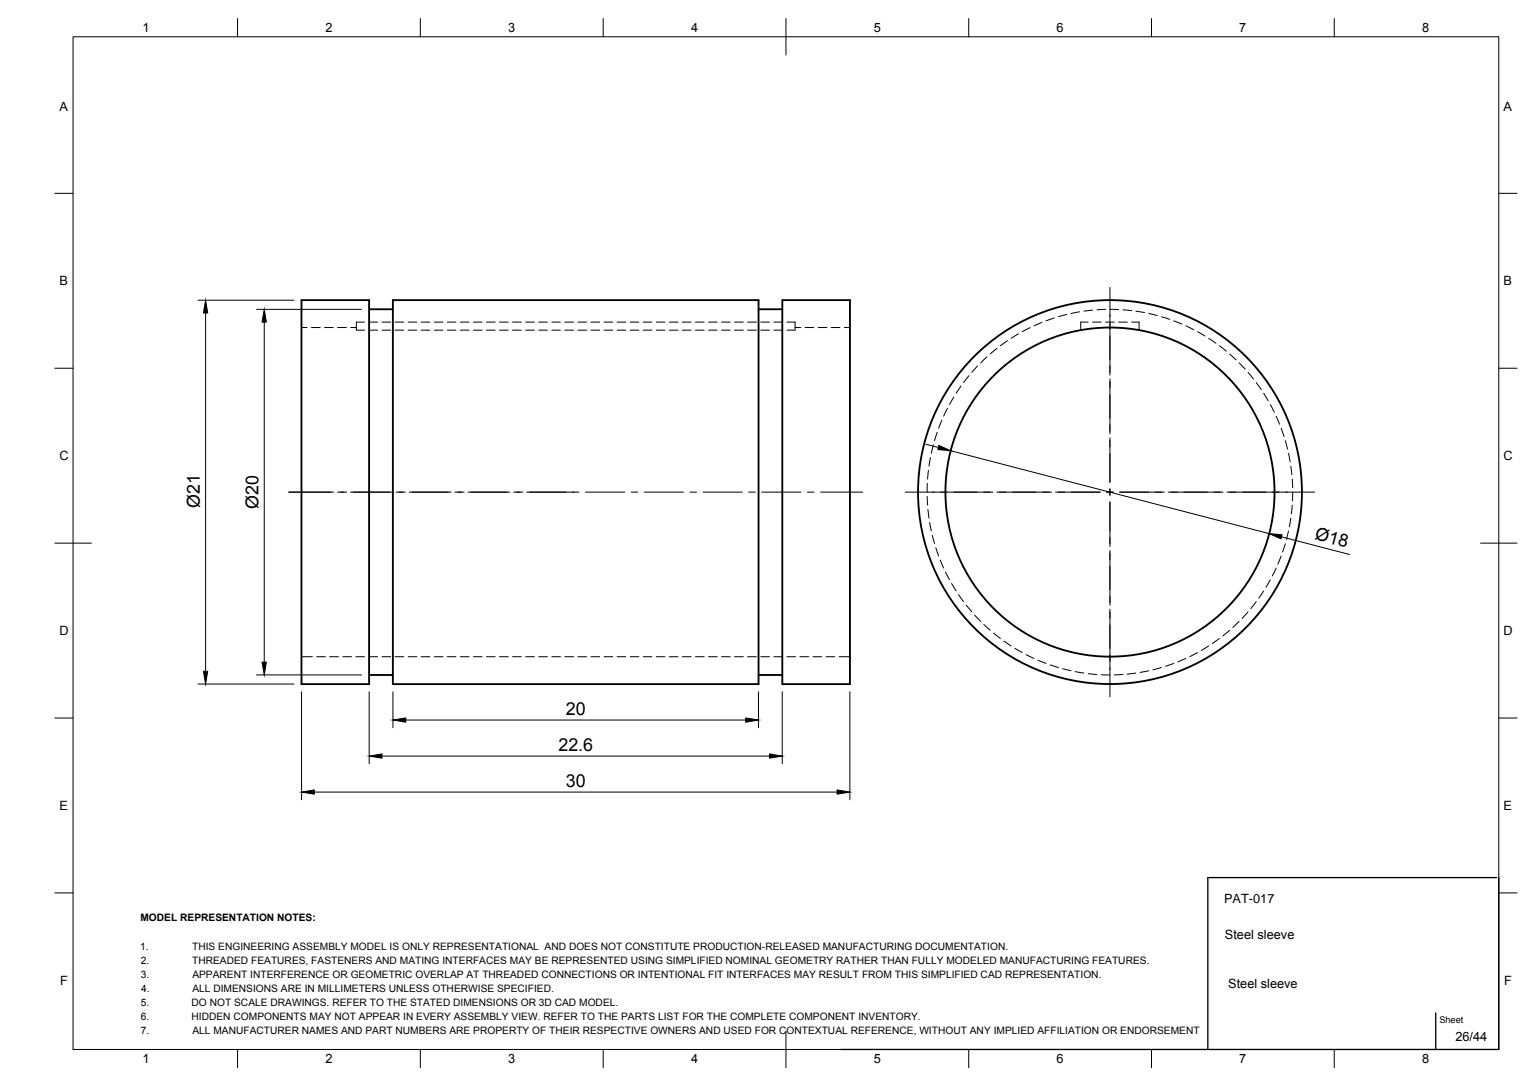
ISO-10303-21;
HEADER;
/* Generated by software containing ST-Developer
 * from STEP Tools, Inc. (www.steptools.com) 
 */

FILE_DESCRIPTION(
/* description */ ('Cam-and-follower valve demonstrator'),
/* implementation_level */ '2;1');

FILE_NAME(
/* name */ 'Steel sleeve.step',
/* time_stamp */ '2026-10-28T03:25:17-07:00',
/* author */ (''),
/* organization */ (''),
/* preprocessor_version */ 'ST-DEVELOPER v20.2',
/* originating_system */ 'Autodesk Translation Framework v15.17.0.0',
/* authorisation */ '');

FILE_SCHEMA (('AUTOMOTIVE_DESIGN { 1 0 10303 214 3 1 1 }'));
ENDSEC;

DATA;
#10=MECHANICAL_DESIGN_GEOMETRIC_PRESENTATION_REPRESENTATION('',(#437),#12896);
#358=SHAPE_REPRESENTATION_RELATIONSHIP('SRR','None',#13076,#394);
#394=ADVANCED_BREP_SHAPE_REPRESENTATION('',(#479),#12876);
#437=STYLED_ITEM('',(#13344),#479);
#479=MANIFOLD_SOLID_BREP('Body1',#6205);
#614=FACE_BOUND('',#1800,.T.);
#615=FACE_BOUND('',#1803,.T.);
#616=FACE_BOUND('',#1806,.T.);
#617=FACE_BOUND('',#1809,.T.);
#618=FACE_BOUND('',#1812,.T.);
#619=FACE_BOUND('',#1815,.T.);
#620=FACE_BOUND('',#1817,.T.);
#868=CIRCLE('',#7071,0.9);
#869=CIRCLE('',#7074,0.9);
#870=CIRCLE('',#7078,1.05);
#871=CIRCLE('',#7079,0.9);
#872=CIRCLE('',#7081,1.05);
#873=CIRCLE('',#7083,1.);
#874=CIRCLE('',#7085,1.);
#875=CIRCLE('',#7087,1.05);
#876=CIRCLE('',#7089,1.05);
#877=CIRCLE('',#7091,1.);
#878=CIRCLE('',#7093,1.);
#879=CIRCLE('',#7095,1.05);
#880=CIRCLE('',#7097,1.05);
#881=CIRCLE('',#7099,0.9);
#1052=CYLINDRICAL_SURFACE('',#7080,1.05);
#1053=CYLINDRICAL_SURFACE('',#7084,1.);
#1054=CYLINDRICAL_SURFACE('',#7088,1.05);
#1055=CYLINDRICAL_SURFACE('',#7092,1.);
#1056=CYLINDRICAL_SURFACE('',#7096,1.05);
#1057=CYLINDRICAL_SURFACE('',#7100,0.9);
#1307=FACE_OUTER_BOUND('',#1794,.T.);
#1308=FACE_OUTER_BOUND('',#1795,.T.);
#1309=FACE_OUTER_BOUND('',#1796,.T.);
#1310=FACE_OUTER_BOUND('',#1797,.T.);
#1311=FACE_OUTER_BOUND('',#1798,.T.);
#1312=FACE_OUTER_BOUND('',#1799,.T.);
#1313=FACE_OUTER_BOUND('',#1801,.T.);
#1314=FACE_OUTER_BOUND('',#1802,.T.);
#1315=FACE_OUTER_BOUND('',#1804,.T.);
#1316=FACE_OUTER_BOUND('',#1805,.T.);
#1317=FACE_OUTER_BOUND('',#1807,.T.);
#1318=FACE_OUTER_BOUND('',#1808,.T.);
#1319=FACE_OUTER_BOUND('',#1810,.T.);
#1320=FACE_OUTER_BOUND('',#1811,.T.);
#1321=FACE_OUTER_BOUND('',#1813,.T.);
#1322=FACE_OUTER_BOUND('',#1814,.T.);
#1323=FACE_OUTER_BOUND('',#1816,.T.);
#1794=EDGE_LOOP('',(#5017,#5018,#5019,#5020));
#1795=EDGE_LOOP('',(#5021,#5022,#5023,#5024));
#1796=EDGE_LOOP('',(#5025,#5026,#5027,#5028));
#1797=EDGE_LOOP('',(#5029,#5030,#5031,#5032));
#1798=EDGE_LOOP('',(#5033,#5034,#5035,#5036));
#1799=EDGE_LOOP('',(#5037));
#1800=EDGE_LOOP('',(#5038));
#1801=EDGE_LOOP('',(#5039,#5040,#5041,#5042));
#1802=EDGE_LOOP('',(#5043));
#1803=EDGE_LOOP('',(#5044));
#1804=EDGE_LOOP('',(#5045,#5046,#5047,#5048));
#1805=EDGE_LOOP('',(#5049));
#1806=EDGE_LOOP('',(#5050));
#1807=EDGE_LOOP('',(#5051,#5052,#5053,#5054));
#1808=EDGE_LOOP('',(#5055));
#1809=EDGE_LOOP('',(#5056));
#1810=EDGE_LOOP('',(#5057,#5058,#5059,#5060));
#1811=EDGE_LOOP('',(#5061));
#1812=EDGE_LOOP('',(#5062));
#1813=EDGE_LOOP('',(#5063,#5064,#5065,#5066));
#1814=EDGE_LOOP('',(#5067));
#1815=EDGE_LOOP('',(#5068));
#1816=EDGE_LOOP('',(#5069,#5070,#5071,#5072));
#1817=EDGE_LOOP('',(#5073,#5074,#5075,#5076));
#2232=LINE('',#12096,#2654);
#2233=LINE('',#12098,#2655);
#2234=LINE('',#12099,#2656);
#2235=LINE('',#12102,#2657);
#2236=LINE('',#12104,#2658);
#2237=LINE('',#12105,#2659);
#2238=LINE('',#12110,#2660);
#2239=LINE('',#12111,#2661);
#2240=LINE('',#12113,#2662);
#2241=LINE('',#12114,#2663);
#2242=LINE('',#12124,#2664);
#2243=LINE('',#12131,#2665);
#2244=LINE('',#12138,#2666);
#2245=LINE('',#12145,#2667);
#2246=LINE('',#12152,#2668);
#2247=LINE('',#12157,#2669);
#2654=VECTOR('',#8551,1.);
#2655=VECTOR('',#8552,1.);
#2656=VECTOR('',#8553,1.);
#2657=VECTOR('',#8556,1.);
#2658=VECTOR('',#8557,1.);
#2659=VECTOR('',#8558,1.);
#2660=VECTOR('',#8563,1.);
#2661=VECTOR('',#8564,1.);
#2662=VECTOR('',#8567,1.);
#2663=VECTOR('',#8568,1.);
#2664=VECTOR('',#8581,1.05);
#2665=VECTOR('',#8590,1.);
#2666=VECTOR('',#8599,1.05);
#2667=VECTOR('',#8608,1.);
#2668=VECTOR('',#8617,1.05);
#2669=VECTOR('',#8624,0.9);
#3153=VERTEX_POINT('',#12092);
#3154=VERTEX_POINT('',#12093);
#3155=VERTEX_POINT('',#12095);
#3156=VERTEX_POINT('',#12097);
#3157=VERTEX_POINT('',#12101);
#3158=VERTEX_POINT('',#12103);
#3159=VERTEX_POINT('',#12107);
#3160=VERTEX_POINT('',#12109);
#3161=VERTEX_POINT('',#12117);
#3162=VERTEX_POINT('',#12119);
#3163=VERTEX_POINT('',#12122);
#3164=VERTEX_POINT('',#12126);
#3165=VERTEX_POINT('',#12129);
#3166=VERTEX_POINT('',#12133);
#3167=VERTEX_POINT('',#12136);
#3168=VERTEX_POINT('',#12140);
#3169=VERTEX_POINT('',#12143);
#3170=VERTEX_POINT('',#12147);
#3171=VERTEX_POINT('',#12150);
#3172=VERTEX_POINT('',#12154);
#3805=EDGE_CURVE('',#3153,#3154,#868,.T.);
#3806=EDGE_CURVE('',#3155,#3153,#2232,.T.);
#3807=EDGE_CURVE('',#3156,#3155,#2233,.T.);
#3808=EDGE_CURVE('',#3154,#3156,#2234,.T.);
#3809=EDGE_CURVE('',#3154,#3157,#2235,.T.);
#3810=EDGE_CURVE('',#3158,#3156,#2236,.T.);
#3811=EDGE_CURVE('',#3158,#3157,#2237,.T.);
#3812=EDGE_CURVE('',#3157,#3159,#869,.T.);
#3813=EDGE_CURVE('',#3160,#3158,#2238,.T.);
#3814=EDGE_CURVE('',#3159,#3160,#2239,.T.);
#3815=EDGE_CURVE('',#3159,#3153,#2240,.T.);
#3816=EDGE_CURVE('',#3160,#3155,#2241,.T.);
#3817=EDGE_CURVE('',#3161,#3161,#870,.T.);
#3818=EDGE_CURVE('',#3162,#3162,#871,.T.);
#3819=EDGE_CURVE('',#3163,#3163,#872,.T.);
#3820=EDGE_CURVE('',#3163,#3161,#2242,.T.);
#3821=EDGE_CURVE('',#3164,#3164,#873,.T.);
#3822=EDGE_CURVE('',#3165,#3165,#874,.T.);
#3823=EDGE_CURVE('',#3165,#3164,#2243,.T.);
#3824=EDGE_CURVE('',#3166,#3166,#875,.T.);
#3825=EDGE_CURVE('',#3167,#3167,#876,.T.);
#3826=EDGE_CURVE('',#3167,#3166,#2244,.T.);
#3827=EDGE_CURVE('',#3168,#3168,#877,.T.);
#3828=EDGE_CURVE('',#3169,#3169,#878,.T.);
#3829=EDGE_CURVE('',#3169,#3168,#2245,.T.);
#3830=EDGE_CURVE('',#3170,#3170,#879,.T.);
#3831=EDGE_CURVE('',#3171,#3171,#880,.T.);
#3832=EDGE_CURVE('',#3171,#3170,#2246,.T.);
#3833=EDGE_CURVE('',#3172,#3172,#881,.T.);
#3834=EDGE_CURVE('',#3172,#3162,#2247,.T.);
#5017=ORIENTED_EDGE('',*,*,#3805,.F.);
#5018=ORIENTED_EDGE('',*,*,#3806,.F.);
#5019=ORIENTED_EDGE('',*,*,#3807,.F.);
#5020=ORIENTED_EDGE('',*,*,#3808,.F.);
#5021=ORIENTED_EDGE('',*,*,#3809,.F.);
#5022=ORIENTED_EDGE('',*,*,#3808,.T.);
#5023=ORIENTED_EDGE('',*,*,#3810,.F.);
#5024=ORIENTED_EDGE('',*,*,#3811,.T.);
#5025=ORIENTED_EDGE('',*,*,#3812,.F.);
#5026=ORIENTED_EDGE('',*,*,#3811,.F.);
#5027=ORIENTED_EDGE('',*,*,#3813,.F.);
#5028=ORIENTED_EDGE('',*,*,#3814,.F.);
#5029=ORIENTED_EDGE('',*,*,#3815,.F.);
#5030=ORIENTED_EDGE('',*,*,#3814,.T.);
#5031=ORIENTED_EDGE('',*,*,#3816,.T.);
#5032=ORIENTED_EDGE('',*,*,#3806,.T.);
#5033=ORIENTED_EDGE('',*,*,#3816,.F.);
#5034=ORIENTED_EDGE('',*,*,#3813,.T.);
#5035=ORIENTED_EDGE('',*,*,#3810,.T.);
#5036=ORIENTED_EDGE('',*,*,#3807,.T.);
#5037=ORIENTED_EDGE('',*,*,#3817,.F.);
#5038=ORIENTED_EDGE('',*,*,#3818,.T.);
#5039=ORIENTED_EDGE('',*,*,#3819,.F.);
#5040=ORIENTED_EDGE('',*,*,#3820,.T.);
#5041=ORIENTED_EDGE('',*,*,#3817,.T.);
#5042=ORIENTED_EDGE('',*,*,#3820,.F.);
#5043=ORIENTED_EDGE('',*,*,#3819,.T.);
#5044=ORIENTED_EDGE('',*,*,#3821,.F.);
#5045=ORIENTED_EDGE('',*,*,#3822,.F.);
#5046=ORIENTED_EDGE('',*,*,#3823,.T.);
#5047=ORIENTED_EDGE('',*,*,#3821,.T.);
#5048=ORIENTED_EDGE('',*,*,#3823,.F.);
#5049=ORIENTED_EDGE('',*,*,#3824,.F.);
#5050=ORIENTED_EDGE('',*,*,#3822,.T.);
#5051=ORIENTED_EDGE('',*,*,#3825,.F.);
#5052=ORIENTED_EDGE('',*,*,#3826,.T.);
#5053=ORIENTED_EDGE('',*,*,#3824,.T.);
#5054=ORIENTED_EDGE('',*,*,#3826,.F.);
#5055=ORIENTED_EDGE('',*,*,#3825,.T.);
#5056=ORIENTED_EDGE('',*,*,#3827,.F.);
#5057=ORIENTED_EDGE('',*,*,#3828,.F.);
#5058=ORIENTED_EDGE('',*,*,#3829,.T.);
#5059=ORIENTED_EDGE('',*,*,#3827,.T.);
#5060=ORIENTED_EDGE('',*,*,#3829,.F.);
#5061=ORIENTED_EDGE('',*,*,#3830,.F.);
#5062=ORIENTED_EDGE('',*,*,#3828,.T.);
#5063=ORIENTED_EDGE('',*,*,#3831,.F.);
#5064=ORIENTED_EDGE('',*,*,#3832,.T.);
#5065=ORIENTED_EDGE('',*,*,#3830,.T.);
#5066=ORIENTED_EDGE('',*,*,#3832,.F.);
#5067=ORIENTED_EDGE('',*,*,#3831,.T.);
#5068=ORIENTED_EDGE('',*,*,#3833,.F.);
#5069=ORIENTED_EDGE('',*,*,#3833,.T.);
#5070=ORIENTED_EDGE('',*,*,#3834,.T.);
#5071=ORIENTED_EDGE('',*,*,#3818,.F.);
#5072=ORIENTED_EDGE('',*,*,#3834,.F.);
#5073=ORIENTED_EDGE('',*,*,#3812,.T.);
#5074=ORIENTED_EDGE('',*,*,#3815,.T.);
#5075=ORIENTED_EDGE('',*,*,#3805,.T.);
#5076=ORIENTED_EDGE('',*,*,#3809,.T.);
#5705=PLANE('',#7070);
#5706=PLANE('',#7072);
#5707=PLANE('',#7073);
#5708=PLANE('',#7075);
#5709=PLANE('',#7076);
#5710=PLANE('',#7077);
#5711=PLANE('',#7082);
#5712=PLANE('',#7086);
#5713=PLANE('',#7090);
#5714=PLANE('',#7094);
#5715=PLANE('',#7098);
#6023=ADVANCED_FACE('',(#1307),#5705,.F.);
#6024=ADVANCED_FACE('',(#1308),#5706,.F.);
#6025=ADVANCED_FACE('',(#1309),#5707,.F.);
#6026=ADVANCED_FACE('',(#1310),#5708,.F.);
#6027=ADVANCED_FACE('',(#1311),#5709,.F.);
#6028=ADVANCED_FACE('',(#1312,#614),#5710,.T.);
#6029=ADVANCED_FACE('',(#1313),#1052,.T.);
#6030=ADVANCED_FACE('',(#1314,#615),#5711,.T.);
#6031=ADVANCED_FACE('',(#1315),#1053,.T.);
#6032=ADVANCED_FACE('',(#1316,#616),#5712,.T.);
#6033=ADVANCED_FACE('',(#1317),#1054,.T.);
#6034=ADVANCED_FACE('',(#1318,#617),#5713,.T.);
#6035=ADVANCED_FACE('',(#1319),#1055,.T.);
#6036=ADVANCED_FACE('',(#1320,#618),#5714,.T.);
#6037=ADVANCED_FACE('',(#1321),#1056,.T.);
#6038=ADVANCED_FACE('',(#1322,#619),#5715,.T.);
#6039=ADVANCED_FACE('',(#1323,#620),#1057,.F.);
#6205=CLOSED_SHELL('',(#6023,#6024,#6025,#6026,#6027,#6028,#6029,#6030,
#6031,#6032,#6033,#6034,#6035,#6036,#6037,#6038,#6039));
#7069=AXIS2_PLACEMENT_3D('',#12090,#8545,#8546);
#7070=AXIS2_PLACEMENT_3D('',#12091,#8547,#8548);
#7071=AXIS2_PLACEMENT_3D('',#12094,#8549,#8550);
#7072=AXIS2_PLACEMENT_3D('',#12100,#8554,#8555);
#7073=AXIS2_PLACEMENT_3D('',#12106,#8559,#8560);
#7074=AXIS2_PLACEMENT_3D('',#12108,#8561,#8562);
#7075=AXIS2_PLACEMENT_3D('',#12112,#8565,#8566);
#7076=AXIS2_PLACEMENT_3D('',#12115,#8569,#8570);
#7077=AXIS2_PLACEMENT_3D('',#12116,#8571,#8572);
#7078=AXIS2_PLACEMENT_3D('',#12118,#8573,#8574);
#7079=AXIS2_PLACEMENT_3D('',#12120,#8575,#8576);
#7080=AXIS2_PLACEMENT_3D('',#12121,#8577,#8578);
#7081=AXIS2_PLACEMENT_3D('',#12123,#8579,#8580);
#7082=AXIS2_PLACEMENT_3D('',#12125,#8582,#8583);
#7083=AXIS2_PLACEMENT_3D('',#12127,#8584,#8585);
#7084=AXIS2_PLACEMENT_3D('',#12128,#8586,#8587);
#7085=AXIS2_PLACEMENT_3D('',#12130,#8588,#8589);
#7086=AXIS2_PLACEMENT_3D('',#12132,#8591,#8592);
#7087=AXIS2_PLACEMENT_3D('',#12134,#8593,#8594);
#7088=AXIS2_PLACEMENT_3D('',#12135,#8595,#8596);
#7089=AXIS2_PLACEMENT_3D('',#12137,#8597,#8598);
#7090=AXIS2_PLACEMENT_3D('',#12139,#8600,#8601);
#7091=AXIS2_PLACEMENT_3D('',#12141,#8602,#8603);
#7092=AXIS2_PLACEMENT_3D('',#12142,#8604,#8605);
#7093=AXIS2_PLACEMENT_3D('',#12144,#8606,#8607);
#7094=AXIS2_PLACEMENT_3D('',#12146,#8609,#8610);
#7095=AXIS2_PLACEMENT_3D('',#12148,#8611,#8612);
#7096=AXIS2_PLACEMENT_3D('',#12149,#8613,#8614);
#7097=AXIS2_PLACEMENT_3D('',#12151,#8615,#8616);
#7098=AXIS2_PLACEMENT_3D('',#12153,#8618,#8619);
#7099=AXIS2_PLACEMENT_3D('',#12155,#8620,#8621);
#7100=AXIS2_PLACEMENT_3D('',#12156,#8622,#8623);
#8545=DIRECTION('axis',(0.,0.,1.));
#8546=DIRECTION('refdir',(1.,0.,0.));
#8547=DIRECTION('center_axis',(0.,1.,0.));
#8548=DIRECTION('ref_axis',(0.,0.,1.));
#8549=DIRECTION('center_axis',(0.,-1.,0.));
#8550=DIRECTION('ref_axis',(1.,0.,0.));
#8551=DIRECTION('',(-1.,0.,0.));
#8552=DIRECTION('',(0.,0.,-1.));
#8553=DIRECTION('',(1.,0.,0.));
#8554=DIRECTION('center_axis',(0.,0.,1.));
#8555=DIRECTION('ref_axis',(1.,0.,0.));
#8556=DIRECTION('',(0.,-1.,0.));
#8557=DIRECTION('',(0.,1.,0.));
#8558=DIRECTION('',(-1.,0.,0.));
#8559=DIRECTION('center_axis',(0.,-1.,0.));
#8560=DIRECTION('ref_axis',(0.,0.,-1.));
#8561=DIRECTION('center_axis',(0.,1.,0.));
#8562=DIRECTION('ref_axis',(1.,0.,0.));
#8563=DIRECTION('',(0.,0.,1.));
#8564=DIRECTION('',(1.,0.,0.));
#8565=DIRECTION('center_axis',(0.,0.,-1.));
#8566=DIRECTION('ref_axis',(-1.,0.,0.));
#8567=DIRECTION('',(0.,1.,0.));
#8568=DIRECTION('',(0.,1.,0.));
#8569=DIRECTION('center_axis',(1.,0.,0.));
#8570=DIRECTION('ref_axis',(0.,0.,-1.));
#8571=DIRECTION('center_axis',(0.,1.,0.));
#8572=DIRECTION('ref_axis',(0.,0.,1.));
#8573=DIRECTION('center_axis',(0.,-1.,0.));
#8574=DIRECTION('ref_axis',(1.,0.,0.));
#8575=DIRECTION('center_axis',(0.,-1.,0.));
#8576=DIRECTION('ref_axis',(1.,0.,0.));
#8577=DIRECTION('center_axis',(0.,-1.,0.));
#8578=DIRECTION('ref_axis',(1.,0.,0.));
#8579=DIRECTION('center_axis',(0.,-1.,0.));
#8580=DIRECTION('ref_axis',(1.,0.,0.));
#8581=DIRECTION('',(0.,1.,0.));
#8582=DIRECTION('center_axis',(0.,-1.,0.));
#8583=DIRECTION('ref_axis',(0.,0.,-1.));
#8584=DIRECTION('center_axis',(0.,-1.,0.));
#8585=DIRECTION('ref_axis',(1.,0.,0.));
#8586=DIRECTION('center_axis',(0.,-1.,0.));
#8587=DIRECTION('ref_axis',(1.,0.,0.));
#8588=DIRECTION('center_axis',(0.,-1.,0.));
#8589=DIRECTION('ref_axis',(1.,0.,0.));
#8590=DIRECTION('',(0.,1.,0.));
#8591=DIRECTION('center_axis',(0.,1.,0.));
#8592=DIRECTION('ref_axis',(0.,0.,1.));
#8593=DIRECTION('center_axis',(0.,-1.,0.));
#8594=DIRECTION('ref_axis',(1.,0.,0.));
#8595=DIRECTION('center_axis',(0.,-1.,0.));
#8596=DIRECTION('ref_axis',(1.,0.,0.));
#8597=DIRECTION('center_axis',(0.,-1.,0.));
#8598=DIRECTION('ref_axis',(1.,0.,0.));
#8599=DIRECTION('',(0.,1.,0.));
#8600=DIRECTION('center_axis',(0.,-1.,0.));
#8601=DIRECTION('ref_axis',(0.,0.,-1.));
#8602=DIRECTION('center_axis',(0.,-1.,0.));
#8603=DIRECTION('ref_axis',(1.,0.,0.));
#8604=DIRECTION('center_axis',(0.,-1.,0.));
#8605=DIRECTION('ref_axis',(1.,0.,0.));
#8606=DIRECTION('center_axis',(0.,-1.,0.));
#8607=DIRECTION('ref_axis',(1.,0.,0.));
#8608=DIRECTION('',(0.,1.,0.));
#8609=DIRECTION('center_axis',(0.,1.,0.));
#8610=DIRECTION('ref_axis',(0.,0.,1.));
#8611=DIRECTION('center_axis',(0.,-1.,0.));
#8612=DIRECTION('ref_axis',(1.,0.,0.));
#8613=DIRECTION('center_axis',(0.,-1.,0.));
#8614=DIRECTION('ref_axis',(1.,0.,0.));
#8615=DIRECTION('center_axis',(0.,-1.,0.));
#8616=DIRECTION('ref_axis',(1.,0.,0.));
#8617=DIRECTION('',(0.,1.,0.));
#8618=DIRECTION('center_axis',(0.,-1.,0.));
#8619=DIRECTION('ref_axis',(0.,0.,-1.));
#8620=DIRECTION('center_axis',(0.,-1.,0.));
#8621=DIRECTION('ref_axis',(1.,0.,0.));
#8622=DIRECTION('center_axis',(0.,-1.,0.));
#8623=DIRECTION('ref_axis',(1.,0.,0.));
#8624=DIRECTION('',(0.,1.,0.));
#12090=CARTESIAN_POINT('',(0.,0.,0.));
#12091=CARTESIAN_POINT('Origin',(0.75,1.2,0.));
#12092=CARTESIAN_POINT('',(0.885663593019381,1.2,-0.16));
#12093=CARTESIAN_POINT('',(0.885663593019381,1.2,0.16));
#12094=CARTESIAN_POINT('Origin',(0.,1.2,0.));
#12095=CARTESIAN_POINT('',(0.93,1.2,-0.16));
#12096=CARTESIAN_POINT('',(0.93,1.2,-0.16));
#12097=CARTESIAN_POINT('',(0.93,1.2,0.16));
#12098=CARTESIAN_POINT('',(0.93,1.2,0.16));
#12099=CARTESIAN_POINT('',(0.57,1.2,0.16));
#12100=CARTESIAN_POINT('Origin',(0.57,0.,0.16));
#12101=CARTESIAN_POINT('',(0.885663593019381,-1.2,0.16));
#12102=CARTESIAN_POINT('',(0.885663593019381,0.,0.16));
#12103=CARTESIAN_POINT('',(0.93,-1.2,0.16));
#12104=CARTESIAN_POINT('',(0.93,0.,0.16));
#12105=CARTESIAN_POINT('',(0.57,-1.2,0.16));
#12106=CARTESIAN_POINT('Origin',(0.75,-1.2,0.));
#12107=CARTESIAN_POINT('',(0.885663593019381,-1.2,-0.16));
#12108=CARTESIAN_POINT('Origin',(0.,-1.2,0.));
#12109=CARTESIAN_POINT('',(0.93,-1.2,-0.16));
#12110=CARTESIAN_POINT('',(0.93,-1.2,0.16));
#12111=CARTESIAN_POINT('',(0.93,-1.2,-0.16));
#12112=CARTESIAN_POINT('Origin',(0.93,0.,-0.16));
#12113=CARTESIAN_POINT('',(0.885663593019381,0.,-0.16));
#12114=CARTESIAN_POINT('',(0.93,0.,-0.16));
#12115=CARTESIAN_POINT('Origin',(0.93,0.,0.16));
#12116=CARTESIAN_POINT('Origin',(1.05,1.5,0.));
#12117=CARTESIAN_POINT('',(-1.05,1.5,-1.28587913910472E-16));
#12118=CARTESIAN_POINT('Origin',(0.,1.5,0.));
#12119=CARTESIAN_POINT('',(-0.9,1.5,-1.10218211923262E-16));
#12120=CARTESIAN_POINT('Origin',(0.,1.5,0.));
#12121=CARTESIAN_POINT('Origin',(0.,1.315,0.));
#12122=CARTESIAN_POINT('',(-1.05,1.13,-1.28587913910472E-16));
#12123=CARTESIAN_POINT('Origin',(0.,1.13,0.));
#12124=CARTESIAN_POINT('',(-1.05,1.315,-1.28587913910472E-16));
#12125=CARTESIAN_POINT('Origin',(1.,1.13,0.));
#12126=CARTESIAN_POINT('',(-1.,1.13,-1.22464679914735E-16));
#12127=CARTESIAN_POINT('Origin',(0.,1.13,0.));
#12128=CARTESIAN_POINT('Origin',(0.,1.065,0.));
#12129=CARTESIAN_POINT('',(-1.,1.,-1.22464679914735E-16));
#12130=CARTESIAN_POINT('Origin',(0.,1.,0.));
#12131=CARTESIAN_POINT('',(-1.,1.065,-1.22464679914735E-16));
#12132=CARTESIAN_POINT('Origin',(1.05,1.,0.));
#12133=CARTESIAN_POINT('',(-1.05,1.,-1.28587913910472E-16));
#12134=CARTESIAN_POINT('Origin',(0.,1.,0.));
#12135=CARTESIAN_POINT('Origin',(0.,0.,0.));
#12136=CARTESIAN_POINT('',(-1.05,-1.,-1.28587913910472E-16));
#12137=CARTESIAN_POINT('Origin',(0.,-1.,0.));
#12138=CARTESIAN_POINT('',(-1.05,0.,-1.28587913910472E-16));
#12139=CARTESIAN_POINT('Origin',(1.,-1.,0.));
#12140=CARTESIAN_POINT('',(-1.,-1.,-1.22464679914735E-16));
#12141=CARTESIAN_POINT('Origin',(0.,-1.,0.));
#12142=CARTESIAN_POINT('Origin',(0.,-1.065,0.));
#12143=CARTESIAN_POINT('',(-1.,-1.13,-1.22464679914735E-16));
#12144=CARTESIAN_POINT('Origin',(0.,-1.13,0.));
#12145=CARTESIAN_POINT('',(-1.,-1.065,-1.22464679914735E-16));
#12146=CARTESIAN_POINT('Origin',(1.05,-1.13,0.));
#12147=CARTESIAN_POINT('',(-1.05,-1.13,-1.28587913910472E-16));
#12148=CARTESIAN_POINT('Origin',(0.,-1.13,0.));
#12149=CARTESIAN_POINT('Origin',(0.,-1.315,0.));
#12150=CARTESIAN_POINT('',(-1.05,-1.5,-1.28587913910472E-16));
#12151=CARTESIAN_POINT('Origin',(0.,-1.5,0.));
#12152=CARTESIAN_POINT('',(-1.05,-1.315,-1.28587913910472E-16));
#12153=CARTESIAN_POINT('Origin',(0.9,-1.5,0.));
#12154=CARTESIAN_POINT('',(-0.9,-1.5,-1.10218211923262E-16));
#12155=CARTESIAN_POINT('Origin',(0.,-1.5,0.));
#12156=CARTESIAN_POINT('Origin',(0.,0.,0.));
#12157=CARTESIAN_POINT('',(-0.9,0.,-1.10218211923262E-16));
#12833=UNCERTAINTY_MEASURE_WITH_UNIT(LENGTH_MEASURE(0.001),#12897,
'DISTANCE_ACCURACY_VALUE',
'Maximum model space distance between geometric entities at asserted c
onnectivities');
#12853=UNCERTAINTY_MEASURE_WITH_UNIT(LENGTH_MEASURE(0.001),#12897,
'DISTANCE_ACCURACY_VALUE',
'Maximum model space distance between geometric entities at asserted c
onnectivities');
#12876=(
GEOMETRIC_REPRESENTATION_CONTEXT(3)
GLOBAL_UNCERTAINTY_ASSIGNED_CONTEXT((#12833))
GLOBAL_UNIT_ASSIGNED_CONTEXT((#12897,#12899,#12900))
REPRESENTATION_CONTEXT('','3D')
);
#12896=(
GEOMETRIC_REPRESENTATION_CONTEXT(3)
GLOBAL_UNCERTAINTY_ASSIGNED_CONTEXT((#12853))
GLOBAL_UNIT_ASSIGNED_CONTEXT((#12897,#12899,#12900))
REPRESENTATION_CONTEXT('','3D')
);
#12897=(
LENGTH_UNIT()
NAMED_UNIT(*)
SI_UNIT(.CENTI.,.METRE.)
);
#12899=(
NAMED_UNIT(*)
PLANE_ANGLE_UNIT()
SI_UNIT($,.RADIAN.)
);
#12900=(
NAMED_UNIT(*)
SI_UNIT($,.STERADIAN.)
SOLID_ANGLE_UNIT()
);
#12923=SHAPE_DEFINITION_REPRESENTATION(#12970,#13076);
#12970=PRODUCT_DEFINITION_SHAPE('',$,#13119);
#13076=SHAPE_REPRESENTATION('',(#7069),#12876);
#13096=PRODUCT_DEFINITION_CONTEXT('part definition',#13224,'design');
#13119=PRODUCT_DEFINITION('Steel sleeve','Steel sleeve',#13161,#13096);
#13161=PRODUCT_DEFINITION_FORMATION('',$,#13248);
#13224=APPLICATION_CONTEXT(
'Core Data for Automotive Mechanical Design Process');
#13225=PRODUCT_CONTEXT('part definition',#13224,'mechanical');
#13248=PRODUCT('Steel sleeve','Steel sleeve','Steel sleeve',(#13225));
#13338=COLOUR_RGB('Off White',0.89,0.88,0.83);
#13339=FILL_AREA_STYLE_COLOUR('',#13338);
#13340=FILL_AREA_STYLE('',(#13339));
#13341=SURFACE_STYLE_FILL_AREA(#13340);
#13342=SURFACE_SIDE_STYLE('',(#13341));
#13343=SURFACE_STYLE_USAGE(.BOTH.,#13342);
#13344=PRESENTATION_STYLE_ASSIGNMENT((#13343));
ENDSEC;
END-ISO-10303-21;
